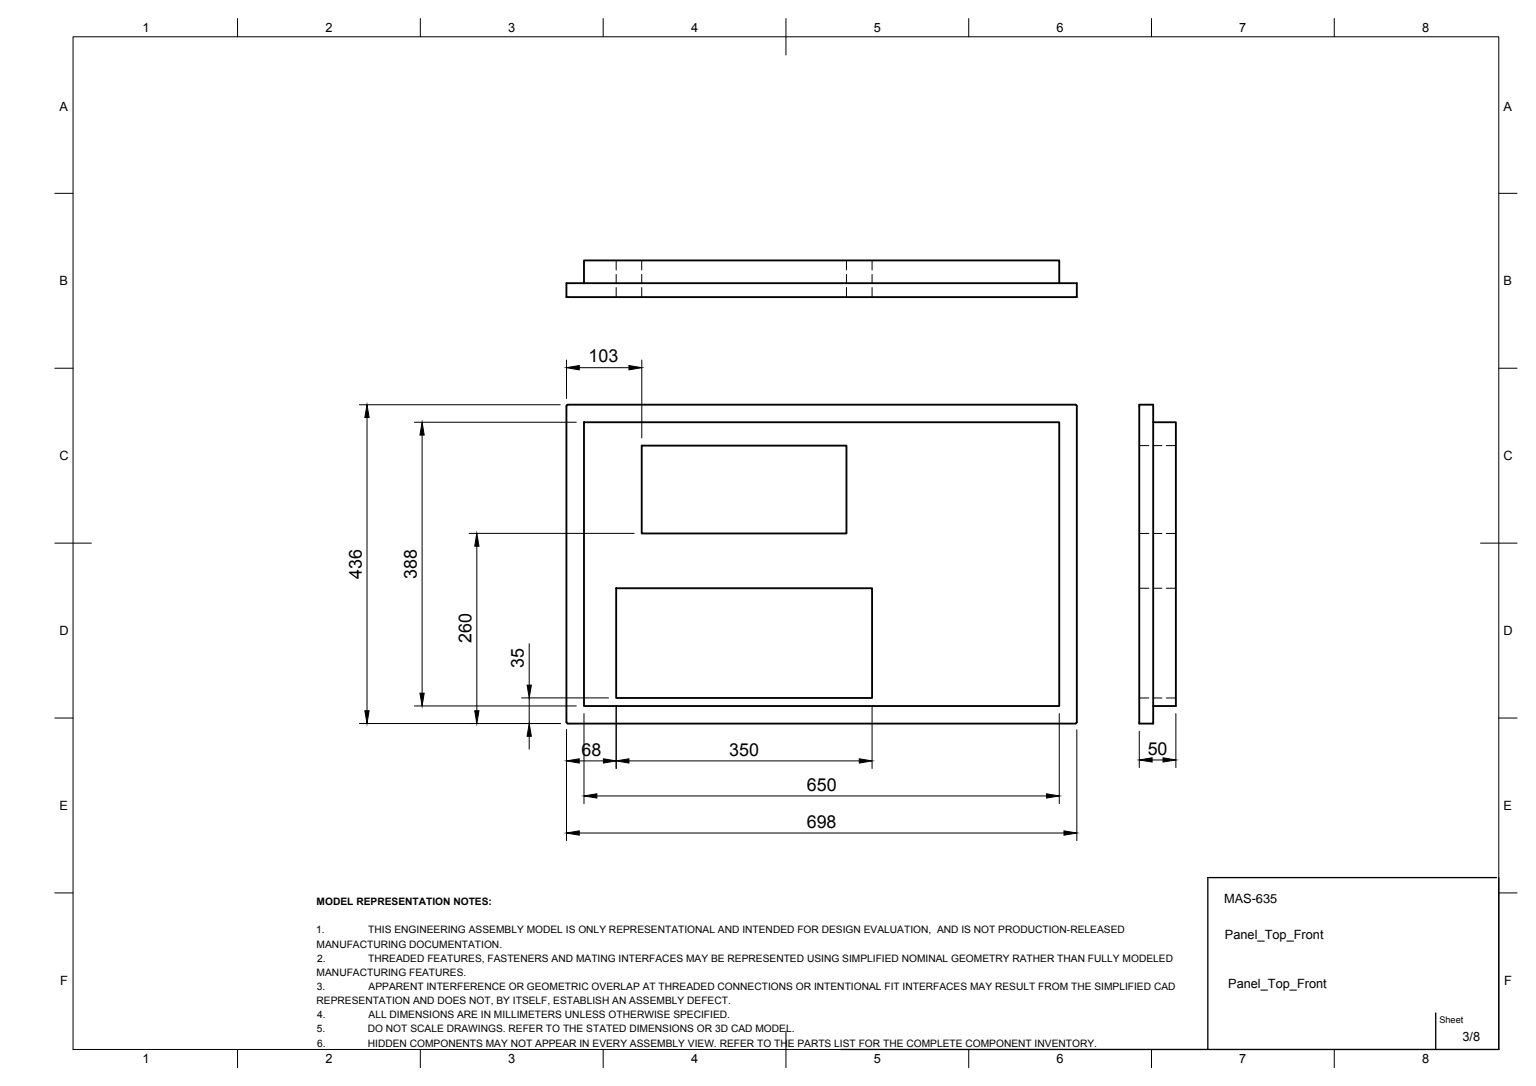
ISO-10303-21;
HEADER;
FILE_DESCRIPTION((''),'2;1');
FILE_NAME('Panel_Top_Front.step','2026-10-09T12:34:24-07:00',(''),(''),'','','');
FILE_SCHEMA (('AUTOMOTIVE_DESIGN { 1 0 10303 214 3 1 1 }'));
ENDSEC;
DATA;
#10=MECHANICAL_DESIGN_GEOMETRIC_PRESENTATION_REPRESENTATION('',(#59),#3759);
#47=SHAPE_REPRESENTATION_RELATIONSHIP('SRR','None',#3788,#53) ;
#53=ADVANCED_BREP_SHAPE_REPRESENTATION('',(#65),#3753) ;
#59=STYLED_ITEM('',(#3827),#65) ;
#65=MANIFOLD_SOLID_BREP('Body1',#2263) ;
#71=CYLINDRICAL_SURFACE('',#2357,0.2) ;
#72=CYLINDRICAL_SURFACE('',#2358,0.2) ;
#73=CYLINDRICAL_SURFACE('',#2359,0.2) ;
#74=CYLINDRICAL_SURFACE('',#2360,0.2) ;
#87=CIRCLE('',#2348,0.2) ;
#88=CIRCLE('',#2349,0.2) ;
#89=CIRCLE('',#2350,0.2) ;
#90=CIRCLE('',#2351,0.2) ;
#91=CIRCLE('',#2353,0.2) ;
#92=CIRCLE('',#2354,0.2) ;
#93=CIRCLE('',#2355,0.2) ;
#94=CIRCLE('',#2356,0.2) ;
#119=FACE_BOUND('',#266,.T.) ;
#120=FACE_BOUND('',#267,.T.) ;
#121=FACE_BOUND('',#273,.T.) ;
#122=FACE_BOUND('',#275,.T.) ;
#123=FACE_BOUND('',#276,.T.) ;
#141=FACE_OUTER_BOUND('',#261,.T.) ;
#142=FACE_OUTER_BOUND('',#262,.T.) ;
#143=FACE_OUTER_BOUND('',#263,.T.) ;
#144=FACE_OUTER_BOUND('',#264,.T.) ;
#145=FACE_OUTER_BOUND('',#265,.T.) ;
#146=FACE_OUTER_BOUND('',#268,.T.) ;
#147=FACE_OUTER_BOUND('',#269,.T.) ;
#148=FACE_OUTER_BOUND('',#270,.T.) ;
#149=FACE_OUTER_BOUND('',#271,.T.) ;
#150=FACE_OUTER_BOUND('',#272,.T.) ;
#151=FACE_OUTER_BOUND('',#274,.T.) ;
#152=FACE_OUTER_BOUND('',#277,.T.) ;
#153=FACE_OUTER_BOUND('',#278,.T.) ;
#154=FACE_OUTER_BOUND('',#279,.T.) ;
#155=FACE_OUTER_BOUND('',#280,.T.) ;
#156=FACE_OUTER_BOUND('',#281,.T.) ;
#157=FACE_OUTER_BOUND('',#282,.T.) ;
#158=FACE_OUTER_BOUND('',#283,.T.) ;
#159=FACE_OUTER_BOUND('',#284,.T.) ;
#160=FACE_OUTER_BOUND('',#285,.T.) ;
#161=FACE_OUTER_BOUND('',#286,.T.) ;
#162=FACE_OUTER_BOUND('',#287,.T.) ;
#163=FACE_OUTER_BOUND('',#288,.T.) ;
#261=EDGE_LOOP('',(#1439,#1440,#1441,#1442)) ;
#262=EDGE_LOOP('',(#1443,#1444,#1445,#1446)) ;
#263=EDGE_LOOP('',(#1447,#1448,#1449,#1450)) ;
#264=EDGE_LOOP('',(#1451,#1452,#1453,#1454)) ;
#265=EDGE_LOOP('',(#1455,#1456,#1457,#1458)) ;
#266=EDGE_LOOP('',(#1459,#1460,#1461,#1462)) ;
#267=EDGE_LOOP('',(#1463,#1464,#1465,#1466)) ;
#268=EDGE_LOOP('',(#1467,#1468,#1469,#1470)) ;
#269=EDGE_LOOP('',(#1471,#1472,#1473,#1474)) ;
#270=EDGE_LOOP('',(#1475,#1476,#1477,#1478)) ;
#271=EDGE_LOOP('',(#1479,#1480,#1481,#1482)) ;
#272=EDGE_LOOP('',(#1483,#1484,#1485,#1486,#1487,#1488,#1489,#1490)) ;
#273=EDGE_LOOP('',(#1491,#1492,#1493,#1494)) ;
#274=EDGE_LOOP('',(#1495,#1496,#1497,#1498,#1499,#1500,#1501,#1502)) ;
#275=EDGE_LOOP('',(#1503,#1504,#1505,#1506)) ;
#276=EDGE_LOOP('',(#1507,#1508,#1509,#1510)) ;
#277=EDGE_LOOP('',(#1511,#1512,#1513,#1514)) ;
#278=EDGE_LOOP('',(#1515,#1516,#1517,#1518)) ;
#279=EDGE_LOOP('',(#1519,#1520,#1521,#1522)) ;
#280=EDGE_LOOP('',(#1523,#1524,#1525,#1526)) ;
#281=EDGE_LOOP('',(#1527,#1528,#1529,#1530)) ;
#282=EDGE_LOOP('',(#1531,#1532,#1533,#1534)) ;
#283=EDGE_LOOP('',(#1535,#1536,#1537,#1538)) ;
#284=EDGE_LOOP('',(#1539,#1540,#1541,#1542)) ;
#285=EDGE_LOOP('',(#1543,#1544,#1545,#1546)) ;
#286=EDGE_LOOP('',(#1547,#1548,#1549,#1550)) ;
#287=EDGE_LOOP('',(#1551,#1552,#1553,#1554)) ;
#288=EDGE_LOOP('',(#1555,#1556,#1557,#1558)) ;
#403=LINE('',#3113,#671) ;
#404=LINE('',#3115,#672) ;
#405=LINE('',#3117,#673) ;
#406=LINE('',#3118,#674) ;
#407=LINE('',#3121,#675) ;
#408=LINE('',#3123,#676) ;
#409=LINE('',#3124,#677) ;
#410=LINE('',#3127,#678) ;
#411=LINE('',#3129,#679) ;
#412=LINE('',#3130,#680) ;
#413=LINE('',#3132,#681) ;
#414=LINE('',#3133,#682) ;
#415=LINE('',#3137,#683) ;
#416=LINE('',#3139,#684) ;
#417=LINE('',#3141,#685) ;
#418=LINE('',#3142,#686) ;
#419=LINE('',#3145,#687) ;
#420=LINE('',#3147,#688) ;
#421=LINE('',#3149,#689) ;
#422=LINE('',#3150,#690) ;
#423=LINE('',#3154,#691) ;
#424=LINE('',#3156,#692) ;
#425=LINE('',#3158,#693) ;
#426=LINE('',#3159,#694) ;
#427=LINE('',#3163,#695) ;
#428=LINE('',#3165,#696) ;
#429=LINE('',#3167,#697) ;
#430=LINE('',#3168,#698) ;
#431=LINE('',#3172,#699) ;
#432=LINE('',#3174,#700) ;
#433=LINE('',#3176,#701) ;
#434=LINE('',#3177,#702) ;
#435=LINE('',#3181,#703) ;
#436=LINE('',#3183,#704) ;
#437=LINE('',#3185,#705) ;
#438=LINE('',#3186,#706) ;
#439=LINE('',#3199,#707) ;
#440=LINE('',#3201,#708) ;
#441=LINE('',#3203,#709) ;
#442=LINE('',#3204,#710) ;
#443=LINE('',#3207,#711) ;
#444=LINE('',#3209,#712) ;
#445=LINE('',#3211,#713) ;
#446=LINE('',#3212,#714) ;
#447=LINE('',#3218,#715) ;
#448=LINE('',#3219,#716) ;
#449=LINE('',#3221,#717) ;
#450=LINE('',#3223,#718) ;
#451=LINE('',#3226,#719) ;
#452=LINE('',#3227,#720) ;
#453=LINE('',#3229,#721) ;
#454=LINE('',#3231,#722) ;
#671=VECTOR('',#2510,100.) ;
#672=VECTOR('',#2511,100.) ;
#673=VECTOR('',#2512,100.) ;
#674=VECTOR('',#2513,100.) ;
#675=VECTOR('',#2516,100.) ;
#676=VECTOR('',#2517,100.) ;
#677=VECTOR('',#2518,100.) ;
#678=VECTOR('',#2521,100.) ;
#679=VECTOR('',#2522,100.) ;
#680=VECTOR('',#2523,100.) ;
#681=VECTOR('',#2526,100.) ;
#682=VECTOR('',#2527,100.) ;
#683=VECTOR('',#2530,100.) ;
#684=VECTOR('',#2531,100.) ;
#685=VECTOR('',#2532,100.) ;
#686=VECTOR('',#2533,100.) ;
#687=VECTOR('',#2534,100.) ;
#688=VECTOR('',#2535,100.) ;
#689=VECTOR('',#2536,100.) ;
#690=VECTOR('',#2537,100.) ;
#691=VECTOR('',#2540,100.) ;
#692=VECTOR('',#2541,100.) ;
#693=VECTOR('',#2542,100.) ;
#694=VECTOR('',#2543,100.) ;
#695=VECTOR('',#2546,100.) ;
#696=VECTOR('',#2547,100.) ;
#697=VECTOR('',#2548,100.) ;
#698=VECTOR('',#2549,100.) ;
#699=VECTOR('',#2552,100.) ;
#700=VECTOR('',#2553,100.) ;
#701=VECTOR('',#2554,100.) ;
#702=VECTOR('',#2555,100.) ;
#703=VECTOR('',#2558,100.) ;
#704=VECTOR('',#2559,100.) ;
#705=VECTOR('',#2560,100.) ;
#706=VECTOR('',#2561,100.) ;
#707=VECTOR('',#2582,100.) ;
#708=VECTOR('',#2583,100.) ;
#709=VECTOR('',#2584,100.) ;
#710=VECTOR('',#2585,100.) ;
#711=VECTOR('',#2586,100.) ;
#712=VECTOR('',#2587,100.) ;
#713=VECTOR('',#2588,100.) ;
#714=VECTOR('',#2589,100.) ;
#715=VECTOR('',#2600,100.) ;
#716=VECTOR('',#2601,100.) ;
#717=VECTOR('',#2604,100.) ;
#718=VECTOR('',#2607,100.) ;
#719=VECTOR('',#2612,100.) ;
#720=VECTOR('',#2613,100.) ;
#721=VECTOR('',#2616,100.) ;
#722=VECTOR('',#2619,100.) ;
#939=VERTEX_POINT('',#3111) ;
#940=VERTEX_POINT('',#3112) ;
#941=VERTEX_POINT('',#3114) ;
#942=VERTEX_POINT('',#3116) ;
#943=VERTEX_POINT('',#3120) ;
#944=VERTEX_POINT('',#3122) ;
#945=VERTEX_POINT('',#3126) ;
#946=VERTEX_POINT('',#3128) ;
#947=VERTEX_POINT('',#3135) ;
#948=VERTEX_POINT('',#3136) ;
#949=VERTEX_POINT('',#3138) ;
#950=VERTEX_POINT('',#3140) ;
#951=VERTEX_POINT('',#3143) ;
#952=VERTEX_POINT('',#3144) ;
#953=VERTEX_POINT('',#3146) ;
#954=VERTEX_POINT('',#3148) ;
#955=VERTEX_POINT('',#3152) ;
#956=VERTEX_POINT('',#3153) ;
#957=VERTEX_POINT('',#3155) ;
#958=VERTEX_POINT('',#3157) ;
#959=VERTEX_POINT('',#3161) ;
#960=VERTEX_POINT('',#3162) ;
#961=VERTEX_POINT('',#3164) ;
#962=VERTEX_POINT('',#3166) ;
#963=VERTEX_POINT('',#3170) ;
#964=VERTEX_POINT('',#3171) ;
#965=VERTEX_POINT('',#3173) ;
#966=VERTEX_POINT('',#3175) ;
#967=VERTEX_POINT('',#3179) ;
#968=VERTEX_POINT('',#3180) ;
#969=VERTEX_POINT('',#3182) ;
#970=VERTEX_POINT('',#3184) ;
#971=VERTEX_POINT('',#3197) ;
#972=VERTEX_POINT('',#3198) ;
#973=VERTEX_POINT('',#3200) ;
#974=VERTEX_POINT('',#3202) ;
#975=VERTEX_POINT('',#3205) ;
#976=VERTEX_POINT('',#3206) ;
#977=VERTEX_POINT('',#3208) ;
#978=VERTEX_POINT('',#3210) ;
#1139=EDGE_CURVE('',#939,#940,#403,.T.) ;
#1140=EDGE_CURVE('',#941,#939,#404,.T.) ;
#1141=EDGE_CURVE('',#941,#942,#405,.T.) ;
#1142=EDGE_CURVE('',#942,#940,#406,.T.) ;
#1143=EDGE_CURVE('',#939,#943,#407,.T.) ;
#1144=EDGE_CURVE('',#944,#943,#408,.T.) ;
#1145=EDGE_CURVE('',#941,#944,#409,.T.) ;
#1146=EDGE_CURVE('',#943,#945,#410,.T.) ;
#1147=EDGE_CURVE('',#946,#945,#411,.T.) ;
#1148=EDGE_CURVE('',#944,#946,#412,.T.) ;
#1149=EDGE_CURVE('',#940,#945,#413,.T.) ;
#1150=EDGE_CURVE('',#942,#946,#414,.T.) ;
#1151=EDGE_CURVE('',#947,#948,#415,.T.) ;
#1152=EDGE_CURVE('',#948,#949,#416,.T.) ;
#1153=EDGE_CURVE('',#949,#950,#417,.T.) ;
#1154=EDGE_CURVE('',#950,#947,#418,.T.) ;
#1155=EDGE_CURVE('',#951,#952,#419,.T.) ;
#1156=EDGE_CURVE('',#952,#953,#420,.T.) ;
#1157=EDGE_CURVE('',#953,#954,#421,.T.) ;
#1158=EDGE_CURVE('',#954,#951,#422,.T.) ;
#1159=EDGE_CURVE('',#955,#956,#423,.T.) ;
#1160=EDGE_CURVE('',#955,#957,#424,.T.) ;
#1161=EDGE_CURVE('',#957,#958,#425,.T.) ;
#1162=EDGE_CURVE('',#958,#956,#426,.T.) ;
#1163=EDGE_CURVE('',#959,#960,#427,.T.) ;
#1164=EDGE_CURVE('',#960,#961,#428,.T.) ;
#1165=EDGE_CURVE('',#962,#961,#429,.T.) ;
#1166=EDGE_CURVE('',#962,#959,#430,.T.) ;
#1167=EDGE_CURVE('',#963,#964,#431,.T.) ;
#1168=EDGE_CURVE('',#963,#965,#432,.T.) ;
#1169=EDGE_CURVE('',#965,#966,#433,.T.) ;
#1170=EDGE_CURVE('',#966,#964,#434,.T.) ;
#1171=EDGE_CURVE('',#967,#968,#435,.T.) ;
#1172=EDGE_CURVE('',#967,#969,#436,.T.) ;
#1173=EDGE_CURVE('',#969,#970,#437,.T.) ;
#1174=EDGE_CURVE('',#970,#968,#438,.T.) ;
#1175=EDGE_CURVE('',#969,#955,#87,.T.) ;
#1176=EDGE_CURVE('',#956,#962,#88,.T.) ;
#1177=EDGE_CURVE('',#961,#966,#89,.T.) ;
#1178=EDGE_CURVE('',#965,#970,#90,.T.) ;
#1179=EDGE_CURVE('',#957,#967,#91,.T.) ;
#1180=EDGE_CURVE('',#968,#963,#92,.T.) ;
#1181=EDGE_CURVE('',#964,#960,#93,.T.) ;
#1182=EDGE_CURVE('',#959,#958,#94,.T.) ;
#1183=EDGE_CURVE('',#971,#972,#439,.T.) ;
#1184=EDGE_CURVE('',#973,#971,#440,.T.) ;
#1185=EDGE_CURVE('',#974,#973,#441,.T.) ;
#1186=EDGE_CURVE('',#972,#974,#442,.T.) ;
#1187=EDGE_CURVE('',#975,#976,#443,.T.) ;
#1188=EDGE_CURVE('',#977,#975,#444,.T.) ;
#1189=EDGE_CURVE('',#978,#977,#445,.T.) ;
#1190=EDGE_CURVE('',#976,#978,#446,.T.) ;
#1191=EDGE_CURVE('',#952,#975,#447,.T.) ;
#1192=EDGE_CURVE('',#953,#976,#448,.T.) ;
#1193=EDGE_CURVE('',#951,#977,#449,.T.) ;
#1194=EDGE_CURVE('',#954,#978,#450,.T.) ;
#1195=EDGE_CURVE('',#948,#971,#451,.T.) ;
#1196=EDGE_CURVE('',#949,#972,#452,.T.) ;
#1197=EDGE_CURVE('',#947,#973,#453,.T.) ;
#1198=EDGE_CURVE('',#950,#974,#454,.T.) ;
#1439=ORIENTED_EDGE('',*,*,#1139,.F.) ;
#1440=ORIENTED_EDGE('',*,*,#1140,.F.) ;
#1441=ORIENTED_EDGE('',*,*,#1141,.T.) ;
#1442=ORIENTED_EDGE('',*,*,#1142,.T.) ;
#1443=ORIENTED_EDGE('',*,*,#1140,.T.) ;
#1444=ORIENTED_EDGE('',*,*,#1143,.T.) ;
#1445=ORIENTED_EDGE('',*,*,#1144,.F.) ;
#1446=ORIENTED_EDGE('',*,*,#1145,.F.) ;
#1447=ORIENTED_EDGE('',*,*,#1144,.T.) ;
#1448=ORIENTED_EDGE('',*,*,#1146,.T.) ;
#1449=ORIENTED_EDGE('',*,*,#1147,.F.) ;
#1450=ORIENTED_EDGE('',*,*,#1148,.F.) ;
#1451=ORIENTED_EDGE('',*,*,#1149,.F.) ;
#1452=ORIENTED_EDGE('',*,*,#1142,.F.) ;
#1453=ORIENTED_EDGE('',*,*,#1150,.T.) ;
#1454=ORIENTED_EDGE('',*,*,#1147,.T.) ;
#1455=ORIENTED_EDGE('',*,*,#1141,.F.) ;
#1456=ORIENTED_EDGE('',*,*,#1145,.T.) ;
#1457=ORIENTED_EDGE('',*,*,#1148,.T.) ;
#1458=ORIENTED_EDGE('',*,*,#1150,.F.) ;
#1459=ORIENTED_EDGE('',*,*,#1151,.T.) ;
#1460=ORIENTED_EDGE('',*,*,#1152,.T.) ;
#1461=ORIENTED_EDGE('',*,*,#1153,.T.) ;
#1462=ORIENTED_EDGE('',*,*,#1154,.T.) ;
#1463=ORIENTED_EDGE('',*,*,#1155,.T.) ;
#1464=ORIENTED_EDGE('',*,*,#1156,.T.) ;
#1465=ORIENTED_EDGE('',*,*,#1157,.T.) ;
#1466=ORIENTED_EDGE('',*,*,#1158,.T.) ;
#1467=ORIENTED_EDGE('',*,*,#1159,.F.) ;
#1468=ORIENTED_EDGE('',*,*,#1160,.T.) ;
#1469=ORIENTED_EDGE('',*,*,#1161,.T.) ;
#1470=ORIENTED_EDGE('',*,*,#1162,.T.) ;
#1471=ORIENTED_EDGE('',*,*,#1163,.T.) ;
#1472=ORIENTED_EDGE('',*,*,#1164,.T.) ;
#1473=ORIENTED_EDGE('',*,*,#1165,.F.) ;
#1474=ORIENTED_EDGE('',*,*,#1166,.T.) ;
#1475=ORIENTED_EDGE('',*,*,#1167,.F.) ;
#1476=ORIENTED_EDGE('',*,*,#1168,.T.) ;
#1477=ORIENTED_EDGE('',*,*,#1169,.T.) ;
#1478=ORIENTED_EDGE('',*,*,#1170,.T.) ;
#1479=ORIENTED_EDGE('',*,*,#1171,.F.) ;
#1480=ORIENTED_EDGE('',*,*,#1172,.T.) ;
#1481=ORIENTED_EDGE('',*,*,#1173,.T.) ;
#1482=ORIENTED_EDGE('',*,*,#1174,.T.) ;
#1483=ORIENTED_EDGE('',*,*,#1173,.F.) ;
#1484=ORIENTED_EDGE('',*,*,#1175,.T.) ;
#1485=ORIENTED_EDGE('',*,*,#1159,.T.) ;
#1486=ORIENTED_EDGE('',*,*,#1176,.T.) ;
#1487=ORIENTED_EDGE('',*,*,#1165,.T.) ;
#1488=ORIENTED_EDGE('',*,*,#1177,.T.) ;
#1489=ORIENTED_EDGE('',*,*,#1169,.F.) ;
#1490=ORIENTED_EDGE('',*,*,#1178,.T.) ;
#1491=ORIENTED_EDGE('',*,*,#1143,.F.) ;
#1492=ORIENTED_EDGE('',*,*,#1139,.T.) ;
#1493=ORIENTED_EDGE('',*,*,#1149,.T.) ;
#1494=ORIENTED_EDGE('',*,*,#1146,.F.) ;
#1495=ORIENTED_EDGE('',*,*,#1161,.F.) ;
#1496=ORIENTED_EDGE('',*,*,#1179,.T.) ;
#1497=ORIENTED_EDGE('',*,*,#1171,.T.) ;
#1498=ORIENTED_EDGE('',*,*,#1180,.T.) ;
#1499=ORIENTED_EDGE('',*,*,#1167,.T.) ;
#1500=ORIENTED_EDGE('',*,*,#1181,.T.) ;
#1501=ORIENTED_EDGE('',*,*,#1163,.F.) ;
#1502=ORIENTED_EDGE('',*,*,#1182,.T.) ;
#1503=ORIENTED_EDGE('',*,*,#1183,.F.) ;
#1504=ORIENTED_EDGE('',*,*,#1184,.F.) ;
#1505=ORIENTED_EDGE('',*,*,#1185,.F.) ;
#1506=ORIENTED_EDGE('',*,*,#1186,.F.) ;
#1507=ORIENTED_EDGE('',*,*,#1187,.F.) ;
#1508=ORIENTED_EDGE('',*,*,#1188,.F.) ;
#1509=ORIENTED_EDGE('',*,*,#1189,.F.) ;
#1510=ORIENTED_EDGE('',*,*,#1190,.F.) ;
#1511=ORIENTED_EDGE('',*,*,#1175,.F.) ;
#1512=ORIENTED_EDGE('',*,*,#1172,.F.) ;
#1513=ORIENTED_EDGE('',*,*,#1179,.F.) ;
#1514=ORIENTED_EDGE('',*,*,#1160,.F.) ;
#1515=ORIENTED_EDGE('',*,*,#1178,.F.) ;
#1516=ORIENTED_EDGE('',*,*,#1168,.F.) ;
#1517=ORIENTED_EDGE('',*,*,#1180,.F.) ;
#1518=ORIENTED_EDGE('',*,*,#1174,.F.) ;
#1519=ORIENTED_EDGE('',*,*,#1177,.F.) ;
#1520=ORIENTED_EDGE('',*,*,#1164,.F.) ;
#1521=ORIENTED_EDGE('',*,*,#1181,.F.) ;
#1522=ORIENTED_EDGE('',*,*,#1170,.F.) ;
#1523=ORIENTED_EDGE('',*,*,#1176,.F.) ;
#1524=ORIENTED_EDGE('',*,*,#1162,.F.) ;
#1525=ORIENTED_EDGE('',*,*,#1182,.F.) ;
#1526=ORIENTED_EDGE('',*,*,#1166,.F.) ;
#1527=ORIENTED_EDGE('',*,*,#1191,.T.) ;
#1528=ORIENTED_EDGE('',*,*,#1187,.T.) ;
#1529=ORIENTED_EDGE('',*,*,#1192,.F.) ;
#1530=ORIENTED_EDGE('',*,*,#1156,.F.) ;
#1531=ORIENTED_EDGE('',*,*,#1193,.T.) ;
#1532=ORIENTED_EDGE('',*,*,#1188,.T.) ;
#1533=ORIENTED_EDGE('',*,*,#1191,.F.) ;
#1534=ORIENTED_EDGE('',*,*,#1155,.F.) ;
#1535=ORIENTED_EDGE('',*,*,#1194,.T.) ;
#1536=ORIENTED_EDGE('',*,*,#1189,.T.) ;
#1537=ORIENTED_EDGE('',*,*,#1193,.F.) ;
#1538=ORIENTED_EDGE('',*,*,#1158,.F.) ;
#1539=ORIENTED_EDGE('',*,*,#1192,.T.) ;
#1540=ORIENTED_EDGE('',*,*,#1190,.T.) ;
#1541=ORIENTED_EDGE('',*,*,#1194,.F.) ;
#1542=ORIENTED_EDGE('',*,*,#1157,.F.) ;
#1543=ORIENTED_EDGE('',*,*,#1195,.T.) ;
#1544=ORIENTED_EDGE('',*,*,#1183,.T.) ;
#1545=ORIENTED_EDGE('',*,*,#1196,.F.) ;
#1546=ORIENTED_EDGE('',*,*,#1152,.F.) ;
#1547=ORIENTED_EDGE('',*,*,#1197,.T.) ;
#1548=ORIENTED_EDGE('',*,*,#1184,.T.) ;
#1549=ORIENTED_EDGE('',*,*,#1195,.F.) ;
#1550=ORIENTED_EDGE('',*,*,#1151,.F.) ;
#1551=ORIENTED_EDGE('',*,*,#1198,.T.) ;
#1552=ORIENTED_EDGE('',*,*,#1185,.T.) ;
#1553=ORIENTED_EDGE('',*,*,#1197,.F.) ;
#1554=ORIENTED_EDGE('',*,*,#1154,.F.) ;
#1555=ORIENTED_EDGE('',*,*,#1196,.T.) ;
#1556=ORIENTED_EDGE('',*,*,#1186,.T.) ;
#1557=ORIENTED_EDGE('',*,*,#1198,.F.) ;
#1558=ORIENTED_EDGE('',*,*,#1153,.F.) ;
#2039=PLANE('',#2338) ;
#2040=PLANE('',#2339) ;
#2041=PLANE('',#2340) ;
#2042=PLANE('',#2341) ;
#2043=PLANE('',#2342) ;
#2044=PLANE('',#2343) ;
#2045=PLANE('',#2344) ;
#2046=PLANE('',#2345) ;
#2047=PLANE('',#2346) ;
#2048=PLANE('',#2347) ;
#2049=PLANE('',#2352) ;
#2050=PLANE('',#2361) ;
#2051=PLANE('',#2362) ;
#2052=PLANE('',#2363) ;
#2053=PLANE('',#2364) ;
#2054=PLANE('',#2365) ;
#2055=PLANE('',#2366) ;
#2056=PLANE('',#2367) ;
#2057=PLANE('',#2368) ;
#2143=ADVANCED_FACE('',(#141),#2039,.T.) ;
#2144=ADVANCED_FACE('',(#142),#2040,.F.) ;
#2145=ADVANCED_FACE('',(#143),#2041,.F.) ;
#2146=ADVANCED_FACE('',(#144),#2042,.T.) ;
#2147=ADVANCED_FACE('',(#145,#119,#120),#2043,.F.) ;
#2148=ADVANCED_FACE('',(#146),#2044,.F.) ;
#2149=ADVANCED_FACE('',(#147),#2045,.F.) ;
#2150=ADVANCED_FACE('',(#148),#2046,.T.) ;
#2151=ADVANCED_FACE('',(#149),#2047,.T.) ;
#2152=ADVANCED_FACE('',(#150,#121),#2048,.T.) ;
#2153=ADVANCED_FACE('',(#151,#122,#123),#2049,.T.) ;
#2154=ADVANCED_FACE('',(#152),#71,.T.) ;
#2155=ADVANCED_FACE('',(#153),#72,.T.) ;
#2156=ADVANCED_FACE('',(#154),#73,.T.) ;
#2157=ADVANCED_FACE('',(#155),#74,.T.) ;
#2158=ADVANCED_FACE('',(#156),#2050,.F.) ;
#2159=ADVANCED_FACE('',(#157),#2051,.F.) ;
#2160=ADVANCED_FACE('',(#158),#2052,.F.) ;
#2161=ADVANCED_FACE('',(#159),#2053,.F.) ;
#2162=ADVANCED_FACE('',(#160),#2054,.F.) ;
#2163=ADVANCED_FACE('',(#161),#2055,.F.) ;
#2164=ADVANCED_FACE('',(#162),#2056,.F.) ;
#2165=ADVANCED_FACE('',(#163),#2057,.F.) ;
#2263=CLOSED_SHELL('',(#2143,#2144,#2145,#2146,#2147,#2148,#2149,#2150,
#2151,#2152,#2153,#2154,#2155,#2156,#2157,#2158,#2159,#2160,#2161,#2162,
#2163,#2164,#2165)) ;
#2337=AXIS2_PLACEMENT_3D('',#3109,#2506,#2507) ;
#2338=AXIS2_PLACEMENT_3D('',#3110,#2508,#2509) ;
#2339=AXIS2_PLACEMENT_3D('',#3119,#2514,#2515) ;
#2340=AXIS2_PLACEMENT_3D('',#3125,#2519,#2520) ;
#2341=AXIS2_PLACEMENT_3D('',#3131,#2524,#2525) ;
#2342=AXIS2_PLACEMENT_3D('',#3134,#2528,#2529) ;
#2343=AXIS2_PLACEMENT_3D('',#3151,#2538,#2539) ;
#2344=AXIS2_PLACEMENT_3D('',#3160,#2544,#2545) ;
#2345=AXIS2_PLACEMENT_3D('',#3169,#2550,#2551) ;
#2346=AXIS2_PLACEMENT_3D('',#3178,#2556,#2557) ;
#2347=AXIS2_PLACEMENT_3D('',#3187,#2562,#2563) ;
#2348=AXIS2_PLACEMENT_3D('',#3188,#2564,#2565) ;
#2349=AXIS2_PLACEMENT_3D('',#3189,#2566,#2567) ;
#2350=AXIS2_PLACEMENT_3D('',#3190,#2568,#2569) ;
#2351=AXIS2_PLACEMENT_3D('',#3191,#2570,#2571) ;
#2352=AXIS2_PLACEMENT_3D('',#3192,#2572,#2573) ;
#2353=AXIS2_PLACEMENT_3D('',#3193,#2574,#2575) ;
#2354=AXIS2_PLACEMENT_3D('',#3194,#2576,#2577) ;
#2355=AXIS2_PLACEMENT_3D('',#3195,#2578,#2579) ;
#2356=AXIS2_PLACEMENT_3D('',#3196,#2580,#2581) ;
#2357=AXIS2_PLACEMENT_3D('',#3213,#2590,#2591) ;
#2358=AXIS2_PLACEMENT_3D('',#3214,#2592,#2593) ;
#2359=AXIS2_PLACEMENT_3D('',#3215,#2594,#2595) ;
#2360=AXIS2_PLACEMENT_3D('',#3216,#2596,#2597) ;
#2361=AXIS2_PLACEMENT_3D('',#3217,#2598,#2599) ;
#2362=AXIS2_PLACEMENT_3D('',#3220,#2602,#2603) ;
#2363=AXIS2_PLACEMENT_3D('',#3222,#2605,#2606) ;
#2364=AXIS2_PLACEMENT_3D('',#3224,#2608,#2609) ;
#2365=AXIS2_PLACEMENT_3D('',#3225,#2610,#2611) ;
#2366=AXIS2_PLACEMENT_3D('',#3228,#2614,#2615) ;
#2367=AXIS2_PLACEMENT_3D('',#3230,#2617,#2618) ;
#2368=AXIS2_PLACEMENT_3D('',#3232,#2620,#2621) ;
#2506=DIRECTION('axis',(0.,0.,1.)) ;
#2507=DIRECTION('refdir',(1.,0.,0.)) ;
#2508=DIRECTION('center_axis',(1.28102656687518E-16,-1.,0.)) ;
#2509=DIRECTION('ref_axis',(1.,1.28102656687518E-16,0.)) ;
#2510=DIRECTION('',(-1.,-1.28102656687518E-16,0.)) ;
#2511=DIRECTION('',(0.,0.,-1.)) ;
#2512=DIRECTION('',(-1.,-1.28102656687518E-16,0.)) ;
#2513=DIRECTION('',(0.,0.,-1.)) ;
#2514=DIRECTION('center_axis',(-1.,0.,0.)) ;
#2515=DIRECTION('ref_axis',(0.,0.,1.)) ;
#2516=DIRECTION('',(0.,1.,0.)) ;
#2517=DIRECTION('',(0.,0.,-1.)) ;
#2518=DIRECTION('',(0.,1.,0.)) ;
#2519=DIRECTION('center_axis',(8.5401771125012E-17,-1.,0.)) ;
#2520=DIRECTION('ref_axis',(1.,8.5401771125012E-17,0.)) ;
#2521=DIRECTION('',(-1.,-8.54017711250121E-17,0.)) ;
#2522=DIRECTION('',(0.,0.,-1.)) ;
#2523=DIRECTION('',(-1.,-8.5401771125012E-17,0.)) ;
#2524=DIRECTION('center_axis',(-1.,0.,0.)) ;
#2525=DIRECTION('ref_axis',(0.,0.,1.)) ;
#2526=DIRECTION('',(0.,1.,0.)) ;
#2527=DIRECTION('',(0.,1.,0.)) ;
#2528=DIRECTION('center_axis',(0.,0.,-1.)) ;
#2529=DIRECTION('ref_axis',(-1.,0.,0.)) ;
#2530=DIRECTION('',(1.,0.,0.)) ;
#2531=DIRECTION('',(0.,-1.,0.)) ;
#2532=DIRECTION('',(-1.,7.43452918275775E-17,0.)) ;
#2533=DIRECTION('',(0.,1.,0.)) ;
#2534=DIRECTION('',(1.,-1.18952466924124E-16,0.)) ;
#2535=DIRECTION('',(0.,-1.,0.)) ;
#2536=DIRECTION('',(-1.,0.,0.)) ;
#2537=DIRECTION('',(0.,1.,0.)) ;
#2538=DIRECTION('center_axis',(-1.,0.,0.)) ;
#2539=DIRECTION('ref_axis',(0.,0.,1.)) ;
#2540=DIRECTION('',(0.,1.,0.)) ;
#2541=DIRECTION('',(0.,0.,-1.)) ;
#2542=DIRECTION('',(0.,1.,0.)) ;
#2543=DIRECTION('',(0.,0.,1.)) ;
#2544=DIRECTION('center_axis',(7.95288699588221E-17,-1.,0.)) ;
#2545=DIRECTION('ref_axis',(1.,7.95288699588221E-17,0.)) ;
#2546=DIRECTION('',(-1.,-7.95288699588221E-17,0.)) ;
#2547=DIRECTION('',(0.,0.,1.)) ;
#2548=DIRECTION('',(-1.,-7.95288699588221E-17,0.)) ;
#2549=DIRECTION('',(0.,0.,-1.)) ;
#2550=DIRECTION('center_axis',(-1.,0.,0.)) ;
#2551=DIRECTION('ref_axis',(0.,0.,1.)) ;
#2552=DIRECTION('',(0.,1.,0.)) ;
#2553=DIRECTION('',(0.,0.,1.)) ;
#2554=DIRECTION('',(0.,1.,0.)) ;
#2555=DIRECTION('',(0.,0.,-1.)) ;
#2556=DIRECTION('center_axis',(1.19293304938233E-16,-1.,0.)) ;
#2557=DIRECTION('ref_axis',(1.,1.19293304938233E-16,0.)) ;
#2558=DIRECTION('',(-1.,-1.19293304938233E-16,0.)) ;
#2559=DIRECTION('',(0.,0.,1.)) ;
#2560=DIRECTION('',(-1.,-1.19293304938233E-16,0.)) ;
#2561=DIRECTION('',(0.,0.,-1.)) ;
#2562=DIRECTION('center_axis',(0.,0.,1.)) ;
#2563=DIRECTION('ref_axis',(1.,0.,0.)) ;
#2564=DIRECTION('center_axis',(0.,0.,1.)) ;
#2565=DIRECTION('ref_axis',(1.,0.,0.)) ;
#2566=DIRECTION('center_axis',(0.,0.,1.)) ;
#2567=DIRECTION('ref_axis',(1.,0.,0.)) ;
#2568=DIRECTION('center_axis',(0.,0.,1.)) ;
#2569=DIRECTION('ref_axis',(1.,0.,0.)) ;
#2570=DIRECTION('center_axis',(0.,0.,1.)) ;
#2571=DIRECTION('ref_axis',(1.,0.,0.)) ;
#2572=DIRECTION('center_axis',(0.,0.,-1.)) ;
#2573=DIRECTION('ref_axis',(-1.,0.,0.)) ;
#2574=DIRECTION('center_axis',(0.,0.,-1.)) ;
#2575=DIRECTION('ref_axis',(-1.,0.,0.)) ;
#2576=DIRECTION('center_axis',(0.,0.,-1.)) ;
#2577=DIRECTION('ref_axis',(-1.,0.,0.)) ;
#2578=DIRECTION('center_axis',(0.,0.,-1.)) ;
#2579=DIRECTION('ref_axis',(-1.,0.,0.)) ;
#2580=DIRECTION('center_axis',(0.,0.,-1.)) ;
#2581=DIRECTION('ref_axis',(-1.,0.,0.)) ;
#2582=DIRECTION('',(0.,-1.,0.)) ;
#2583=DIRECTION('',(1.,0.,0.)) ;
#2584=DIRECTION('',(0.,1.,0.)) ;
#2585=DIRECTION('',(-1.,7.43452918275774E-17,0.)) ;
#2586=DIRECTION('',(0.,-1.,0.)) ;
#2587=DIRECTION('',(1.,-1.18952466924124E-16,0.)) ;
#2588=DIRECTION('',(0.,1.,0.)) ;
#2589=DIRECTION('',(-1.,0.,0.)) ;
#2590=DIRECTION('center_axis',(0.,0.,1.)) ;
#2591=DIRECTION('ref_axis',(1.,0.,0.)) ;
#2592=DIRECTION('center_axis',(0.,0.,-1.)) ;
#2593=DIRECTION('ref_axis',(-1.,0.,0.)) ;
#2594=DIRECTION('center_axis',(0.,0.,1.)) ;
#2595=DIRECTION('ref_axis',(1.,0.,0.)) ;
#2596=DIRECTION('center_axis',(0.,0.,-1.)) ;
#2597=DIRECTION('ref_axis',(-1.,0.,0.)) ;
#2598=DIRECTION('center_axis',(1.,0.,0.)) ;
#2599=DIRECTION('ref_axis',(0.,0.,-1.)) ;
#2600=DIRECTION('',(0.,0.,-1.)) ;
#2601=DIRECTION('',(0.,0.,-1.)) ;
#2602=DIRECTION('center_axis',(1.18952466924124E-16,1.,0.)) ;
#2603=DIRECTION('ref_axis',(-1.,1.18952466924124E-16,0.)) ;
#2604=DIRECTION('',(0.,0.,-1.)) ;
#2605=DIRECTION('center_axis',(-1.,0.,0.)) ;
#2606=DIRECTION('ref_axis',(0.,0.,1.)) ;
#2607=DIRECTION('',(0.,0.,-1.)) ;
#2608=DIRECTION('center_axis',(0.,-1.,0.)) ;
#2609=DIRECTION('ref_axis',(0.,0.,-1.)) ;
#2610=DIRECTION('center_axis',(1.,0.,0.)) ;
#2611=DIRECTION('ref_axis',(0.,0.,-1.)) ;
#2612=DIRECTION('',(0.,0.,-1.)) ;
#2613=DIRECTION('',(0.,0.,-1.)) ;
#2614=DIRECTION('center_axis',(0.,1.,0.)) ;
#2615=DIRECTION('ref_axis',(0.,0.,1.)) ;
#2616=DIRECTION('',(0.,0.,-1.)) ;
#2617=DIRECTION('center_axis',(-1.,0.,0.)) ;
#2618=DIRECTION('ref_axis',(0.,0.,1.)) ;
#2619=DIRECTION('',(0.,0.,-1.)) ;
#2620=DIRECTION('center_axis',(-7.43452918275775E-17,-1.,0.)) ;
#2621=DIRECTION('ref_axis',(1.,-7.43452918275775E-17,0.)) ;
#3109=CARTESIAN_POINT('',(0.,0.,0.)) ;
#3110=CARTESIAN_POINT('Origin',(32.5,-19.4,5.)) ;
#3111=CARTESIAN_POINT('',(32.5,-19.4,1.9)) ;
#3112=CARTESIAN_POINT('',(-32.5,-19.4,1.9)) ;
#3113=CARTESIAN_POINT('',(32.5,-19.4,1.9)) ;
#3114=CARTESIAN_POINT('',(32.5,-19.4,5.)) ;
#3115=CARTESIAN_POINT('',(32.5,-19.4,5.)) ;
#3116=CARTESIAN_POINT('',(-32.5,-19.4,5.)) ;
#3117=CARTESIAN_POINT('',(32.5,-19.4,5.)) ;
#3118=CARTESIAN_POINT('',(-32.5,-19.4,5.)) ;
#3119=CARTESIAN_POINT('Origin',(32.5,-19.4,5.)) ;
#3120=CARTESIAN_POINT('',(32.5,19.4,1.9)) ;
#3121=CARTESIAN_POINT('',(32.5,-19.4,1.9)) ;
#3122=CARTESIAN_POINT('',(32.5,19.4,5.)) ;
#3123=CARTESIAN_POINT('',(32.5,19.4,5.)) ;
#3124=CARTESIAN_POINT('',(32.5,-19.4,5.)) ;
#3125=CARTESIAN_POINT('Origin',(32.5,19.4,5.)) ;
#3126=CARTESIAN_POINT('',(-32.5,19.4,1.9)) ;
#3127=CARTESIAN_POINT('',(32.5,19.4,1.9)) ;
#3128=CARTESIAN_POINT('',(-32.5,19.4,5.)) ;
#3129=CARTESIAN_POINT('',(-32.5,19.4,5.)) ;
#3130=CARTESIAN_POINT('',(32.5,19.4,5.)) ;
#3131=CARTESIAN_POINT('Origin',(-32.5,-19.4,5.)) ;
#3132=CARTESIAN_POINT('',(-32.5,-19.4,1.9)) ;
#3133=CARTESIAN_POINT('',(-32.5,-19.4,5.)) ;
#3134=CARTESIAN_POINT('Origin',(0.,0.,5.)) ;
#3135=CARTESIAN_POINT('',(-24.6,16.2,5.)) ;
#3136=CARTESIAN_POINT('',(3.4,16.2,5.)) ;
#3137=CARTESIAN_POINT('',(0.,16.2,5.)) ;
#3138=CARTESIAN_POINT('',(3.4,4.20000000000001,5.)) ;
#3139=CARTESIAN_POINT('',(3.4,0.,5.)) ;
#3140=CARTESIAN_POINT('',(-24.6,4.20000000000001,5.)) ;
#3141=CARTESIAN_POINT('',(3.12250225675826E-16,4.20000000000001,5.)) ;
#3142=CARTESIAN_POINT('',(-24.6,0.,5.)) ;
#3143=CARTESIAN_POINT('',(-28.1,-3.29999999999999,5.)) ;
#3144=CARTESIAN_POINT('',(6.90000000000001,-3.29999999999999,5.)) ;
#3145=CARTESIAN_POINT('',(-3.92543140849608E-16,-3.29999999999999,5.)) ;
#3146=CARTESIAN_POINT('',(6.90000000000001,-18.3,5.)) ;
#3147=CARTESIAN_POINT('',(6.90000000000001,0.,5.)) ;
#3148=CARTESIAN_POINT('',(-28.1,-18.3,5.)) ;
#3149=CARTESIAN_POINT('',(0.,-18.3,5.)) ;
#3150=CARTESIAN_POINT('',(-28.1,0.,5.)) ;
#3151=CARTESIAN_POINT('Origin',(34.9,-21.8,1.9)) ;
#3152=CARTESIAN_POINT('',(34.9,-21.6,1.9)) ;
#3153=CARTESIAN_POINT('',(34.9,21.6,1.9)) ;
#3154=CARTESIAN_POINT('',(34.9,-21.8,1.9)) ;
#3155=CARTESIAN_POINT('',(34.9,-21.6,0.)) ;
#3156=CARTESIAN_POINT('',(34.9,-21.6,0.)) ;
#3157=CARTESIAN_POINT('',(34.9,21.6,0.)) ;
#3158=CARTESIAN_POINT('',(34.9,-21.8,0.)) ;
#3159=CARTESIAN_POINT('',(34.9,21.6,1.9)) ;
#3160=CARTESIAN_POINT('Origin',(34.9,21.8,1.9)) ;
#3161=CARTESIAN_POINT('',(34.7,21.8,0.)) ;
#3162=CARTESIAN_POINT('',(-34.7,21.8,0.)) ;
#3163=CARTESIAN_POINT('',(34.9,21.8,0.)) ;
#3164=CARTESIAN_POINT('',(-34.7,21.8,1.9)) ;
#3165=CARTESIAN_POINT('',(-34.7,21.8,1.9)) ;
#3166=CARTESIAN_POINT('',(34.7,21.8,1.9)) ;
#3167=CARTESIAN_POINT('',(34.9,21.8,1.9)) ;
#3168=CARTESIAN_POINT('',(34.7,21.8,1.9)) ;
#3169=CARTESIAN_POINT('Origin',(-34.9,-21.8,1.9)) ;
#3170=CARTESIAN_POINT('',(-34.9,-21.6,0.)) ;
#3171=CARTESIAN_POINT('',(-34.9,21.6,0.)) ;
#3172=CARTESIAN_POINT('',(-34.9,-21.8,0.)) ;
#3173=CARTESIAN_POINT('',(-34.9,-21.6,1.9)) ;
#3174=CARTESIAN_POINT('',(-34.9,-21.6,1.9)) ;
#3175=CARTESIAN_POINT('',(-34.9,21.6,1.9)) ;
#3176=CARTESIAN_POINT('',(-34.9,-21.8,1.9)) ;
#3177=CARTESIAN_POINT('',(-34.9,21.6,0.)) ;
#3178=CARTESIAN_POINT('Origin',(34.9,-21.8,1.9)) ;
#3179=CARTESIAN_POINT('',(34.7,-21.8,0.)) ;
#3180=CARTESIAN_POINT('',(-34.7,-21.8,0.)) ;
#3181=CARTESIAN_POINT('',(34.9,-21.8,0.)) ;
#3182=CARTESIAN_POINT('',(34.7,-21.8,1.9)) ;
#3183=CARTESIAN_POINT('',(34.7,-21.8,1.9)) ;
#3184=CARTESIAN_POINT('',(-34.7,-21.8,1.9)) ;
#3185=CARTESIAN_POINT('',(34.9,-21.8,1.9)) ;
#3186=CARTESIAN_POINT('',(-34.7,-21.8,1.9)) ;
#3187=CARTESIAN_POINT('Origin',(0.,0.,1.9)) ;
#3188=CARTESIAN_POINT('Origin',(34.7,-21.6,1.9)) ;
#3189=CARTESIAN_POINT('Origin',(34.7,21.6,1.9)) ;
#3190=CARTESIAN_POINT('Origin',(-34.7,21.6,1.9)) ;
#3191=CARTESIAN_POINT('Origin',(-34.7,-21.6,1.9)) ;
#3192=CARTESIAN_POINT('Origin',(0.,0.,0.)) ;
#3193=CARTESIAN_POINT('Origin',(34.7,-21.6,0.)) ;
#3194=CARTESIAN_POINT('Origin',(-34.7,-21.6,0.)) ;
#3195=CARTESIAN_POINT('Origin',(-34.7,21.6,0.)) ;
#3196=CARTESIAN_POINT('Origin',(34.7,21.6,0.)) ;
#3197=CARTESIAN_POINT('',(3.4,16.2,0.)) ;
#3198=CARTESIAN_POINT('',(3.4,4.20000000000001,0.)) ;
#3199=CARTESIAN_POINT('',(3.4,4.20000000000001,0.)) ;
#3200=CARTESIAN_POINT('',(-24.6,16.2,0.)) ;
#3201=CARTESIAN_POINT('',(-24.6,16.2,0.)) ;
#3202=CARTESIAN_POINT('',(-24.6,4.20000000000001,0.)) ;
#3203=CARTESIAN_POINT('',(-24.6,4.20000000000001,0.)) ;
#3204=CARTESIAN_POINT('',(-24.6,4.20000000000001,0.)) ;
#3205=CARTESIAN_POINT('',(6.90000000000001,-3.29999999999999,0.)) ;
#3206=CARTESIAN_POINT('',(6.90000000000001,-18.3,0.)) ;
#3207=CARTESIAN_POINT('',(6.90000000000001,-18.3,0.)) ;
#3208=CARTESIAN_POINT('',(-28.1,-3.29999999999999,0.)) ;
#3209=CARTESIAN_POINT('',(-28.1,-3.29999999999999,0.)) ;
#3210=CARTESIAN_POINT('',(-28.1,-18.3,0.)) ;
#3211=CARTESIAN_POINT('',(-28.1,-18.3,0.)) ;
#3212=CARTESIAN_POINT('',(-28.1,-18.3,0.)) ;
#3213=CARTESIAN_POINT('Origin',(34.7,-21.6,1.9)) ;
#3214=CARTESIAN_POINT('Origin',(-34.7,-21.6,1.9)) ;
#3215=CARTESIAN_POINT('Origin',(-34.7,21.6,1.9)) ;
#3216=CARTESIAN_POINT('Origin',(34.7,21.6,1.9)) ;
#3217=CARTESIAN_POINT('Origin',(6.90000000000001,-18.3,6.)) ;
#3218=CARTESIAN_POINT('',(6.90000000000001,-3.29999999999999,6.)) ;
#3219=CARTESIAN_POINT('',(6.90000000000001,-18.3,6.)) ;
#3220=CARTESIAN_POINT('Origin',(-28.1,-3.29999999999999,6.)) ;
#3221=CARTESIAN_POINT('',(-28.1,-3.29999999999999,6.)) ;
#3222=CARTESIAN_POINT('Origin',(-28.1,-18.3,6.)) ;
#3223=CARTESIAN_POINT('',(-28.1,-18.3,6.)) ;
#3224=CARTESIAN_POINT('Origin',(-28.1,-18.3,6.)) ;
#3225=CARTESIAN_POINT('Origin',(3.4,4.20000000000001,6.)) ;
#3226=CARTESIAN_POINT('',(3.4,16.2,6.)) ;
#3227=CARTESIAN_POINT('',(3.4,4.20000000000001,6.)) ;
#3228=CARTESIAN_POINT('Origin',(-24.6,16.2,6.)) ;
#3229=CARTESIAN_POINT('',(-24.6,16.2,6.)) ;
#3230=CARTESIAN_POINT('Origin',(-24.6,4.20000000000001,6.)) ;
#3231=CARTESIAN_POINT('',(-24.6,4.20000000000001,6.)) ;
#3232=CARTESIAN_POINT('Origin',(-24.6,4.20000000000001,6.)) ;
#3745=UNCERTAINTY_MEASURE_WITH_UNIT(LENGTH_MEASURE(0.001),#3760,
'DISTANCE_ACCURACY_VALUE',
'Maximum model space distance between geometric entities at asserted c
onnectivities') ;
#3751=UNCERTAINTY_MEASURE_WITH_UNIT(LENGTH_MEASURE(0.001),#3760,
'DISTANCE_ACCURACY_VALUE',
'Maximum model space distance between geometric entities at asserted c
onnectivities') ;
#3753=(
GEOMETRIC_REPRESENTATION_CONTEXT(3)
GLOBAL_UNCERTAINTY_ASSIGNED_CONTEXT((#3745))
GLOBAL_UNIT_ASSIGNED_CONTEXT((#3760,#3762,#3763))
REPRESENTATION_CONTEXT('','3D')
) ;
#3759=(
GEOMETRIC_REPRESENTATION_CONTEXT(3)
GLOBAL_UNCERTAINTY_ASSIGNED_CONTEXT((#3751))
GLOBAL_UNIT_ASSIGNED_CONTEXT((#3760,#3762,#3763))
REPRESENTATION_CONTEXT('','3D')
) ;
#3760=(
LENGTH_UNIT()
NAMED_UNIT(*)
SI_UNIT(.CENTI.,.METRE.)
) ;
#3762=(
NAMED_UNIT(*)
PLANE_ANGLE_UNIT()
SI_UNIT($,.RADIAN.)
) ;
#3763=(
NAMED_UNIT(*)
SI_UNIT($,.STERADIAN.)
SOLID_ANGLE_UNIT()
) ;
#3765=SHAPE_DEFINITION_REPRESENTATION(#3772,#3788) ;
#3772=PRODUCT_DEFINITION_SHAPE('',$,#3796) ;
#3788=SHAPE_REPRESENTATION('',(#2337),#3753) ;
#3794=PRODUCT_DEFINITION_CONTEXT('part definition',#3817,'design') ;
#3796=PRODUCT_DEFINITION('Panel_Top_Front','Panel_Top_Front',
#3803,#3794) ;
#3803=PRODUCT_DEFINITION_FORMATION('',$,#3820) ;
#3817=APPLICATION_CONTEXT(
'Core Data for Automotive Mechanical Design Process') ;
#3818=PRODUCT_CONTEXT('part definition',#3817,'mechanical') ;
#3820=PRODUCT('Panel_Top_Front','Panel_Top_Front',$,(#3818)) ;
#3827=PRESENTATION_STYLE_ASSIGNMENT((#3829)) ;
#3829=SURFACE_STYLE_USAGE(.BOTH.,#3831) ;
#3831=SURFACE_SIDE_STYLE('',(#3833)) ;
#3833=SURFACE_STYLE_FILL_AREA(#3835) ;
#3835=FILL_AREA_STYLE('Opaque(179,179,179)',(#3837)) ;
#3837=FILL_AREA_STYLE_COLOUR('Opaque(179,179,179)',#3839) ;
#3839=COLOUR_RGB('Opaque(179,179,179)', 0.09019608, 0.27058824, 0.51372549) ;
ENDSEC;
END-ISO-10303-21;
